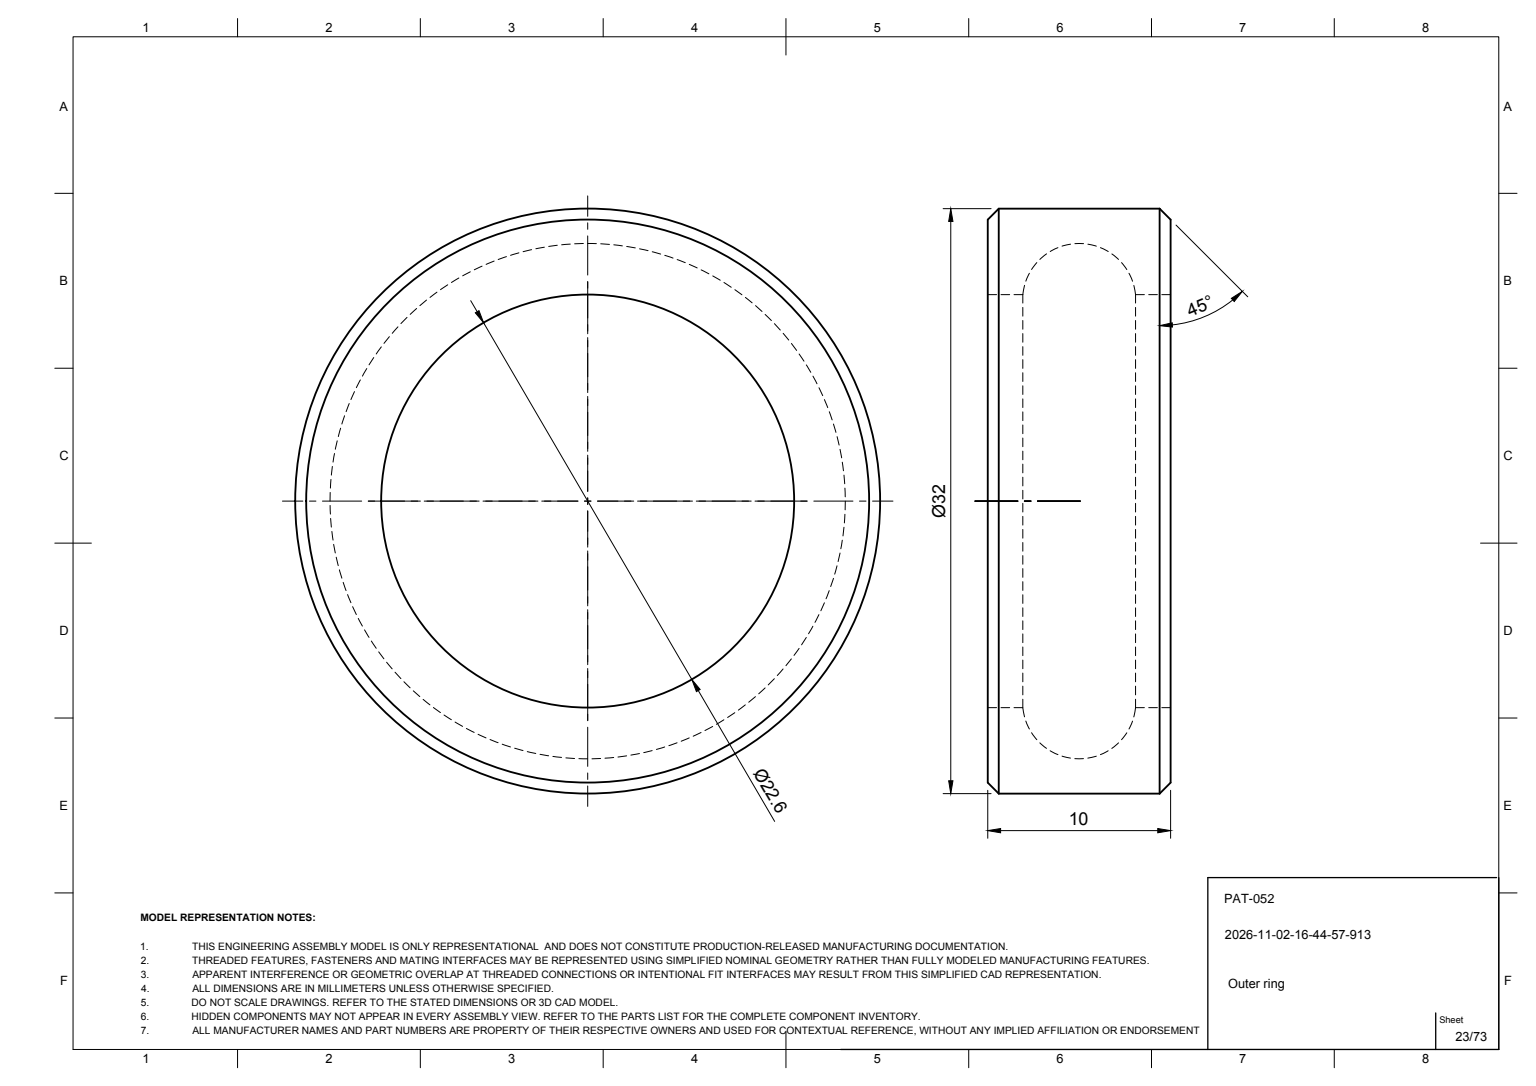
ISO-10303-21;
HEADER;
/* Generated by software containing ST-Developer
 * from STEP Tools, Inc. (www.steptools.com) 
 */

FILE_DESCRIPTION(
/* description */ ('Hand-crank gear train demonstrator'),
/* implementation_level */ '2;1');

FILE_NAME(
/* name */ 'Outer ring.step',
/* time_stamp */ '2026-10-28T03:22:13-07:00',
/* author */ (''),
/* organization */ (''),
/* preprocessor_version */ 'ST-DEVELOPER v20.2',
/* originating_system */ 'Autodesk Translation Framework v15.17.0.0',
/* authorisation */ '');

FILE_SCHEMA (('AUTOMOTIVE_DESIGN { 1 0 10303 214 3 1 1 }'));
ENDSEC;

DATA;
#10=MECHANICAL_DESIGN_GEOMETRIC_PRESENTATION_REPRESENTATION('',(#1201),#62758);
#1022=TOROIDAL_SURFACE('',#17506,1.1,0.309556);
#1030=CONICAL_SURFACE('',#17517,1.57,0.785398163397449);
#1031=CONICAL_SURFACE('',#17521,1.57,0.785398163397449);
#1073=SHAPE_REPRESENTATION_RELATIONSHIP('SRR','None',#63046,#1137);
#1137=ADVANCED_BREP_SHAPE_REPRESENTATION('',(#1279),#62700);
#1201=STYLED_ITEM('',(#63462),#1279);
#1279=MANIFOLD_SOLID_BREP('Body1',#16382);
#1489=FACE_BOUND('',#3355,.T.);
#1490=FACE_BOUND('',#3360,.T.);
#1684=PLANE('',#17514);
#1685=PLANE('',#17523);
#2269=FACE_OUTER_BOUND('',#3352,.T.);
#2270=FACE_OUTER_BOUND('',#3353,.T.);
#2271=FACE_OUTER_BOUND('',#3354,.T.);
#2272=FACE_OUTER_BOUND('',#3356,.T.);
#2273=FACE_OUTER_BOUND('',#3357,.T.);
#2274=FACE_OUTER_BOUND('',#3358,.T.);
#2275=FACE_OUTER_BOUND('',#3359,.T.);
#2276=FACE_OUTER_BOUND('',#3361,.T.);
#3352=EDGE_LOOP('',(#11491,#11492,#11493,#11494,#11495,#11496));
#3353=EDGE_LOOP('',(#11497,#11498,#11499,#11500,#11501));
#3354=EDGE_LOOP('',(#11502));
#3355=EDGE_LOOP('',(#11503));
#3356=EDGE_LOOP('',(#11504,#11505,#11506,#11507));
#3357=EDGE_LOOP('',(#11508,#11509,#11510,#11511));
#3358=EDGE_LOOP('',(#11512,#11513,#11514,#11515));
#3359=EDGE_LOOP('',(#11516));
#3360=EDGE_LOOP('',(#11517));
#3361=EDGE_LOOP('',(#11518,#11519,#11520,#11521,#11522));
#4428=LINE('',#24029,#5560);
#4429=LINE('',#24038,#5561);
#4430=LINE('',#24042,#5562);
#4431=LINE('',#24046,#5563);
#4432=LINE('',#24049,#5564);
#5560=VECTOR('',#19685,1.129765);
#5561=VECTOR('',#19696,1.57);
#5562=VECTOR('',#19701,1.6);
#5563=VECTOR('',#19706,1.57);
#5564=VECTOR('',#19711,1.129765);
#6736=CIRCLE('',#17507,1.129765);
#6737=CIRCLE('',#17508,1.129765);
#6738=CIRCLE('',#17509,0.309556);
#6739=CIRCLE('',#17510,1.129765);
#6740=CIRCLE('',#17511,1.129765);
#6741=CIRCLE('',#17513,1.129765);
#6742=CIRCLE('',#17515,1.54);
#6743=CIRCLE('',#17516,1.129765);
#6744=CIRCLE('',#17518,1.6);
#6745=CIRCLE('',#17520,1.6);
#6746=CIRCLE('',#17522,1.54);
#7429=VERTEX_POINT('',#24017);
#7430=VERTEX_POINT('',#24018);
#7431=VERTEX_POINT('',#24021);
#7432=VERTEX_POINT('',#24023);
#7433=VERTEX_POINT('',#24027);
#7434=VERTEX_POINT('',#24031);
#7435=VERTEX_POINT('',#24033);
#7436=VERTEX_POINT('',#24036);
#7437=VERTEX_POINT('',#24040);
#7438=VERTEX_POINT('',#24044);
#8997=EDGE_CURVE('',#7429,#7430,#6736,.T.);
#8998=EDGE_CURVE('',#7430,#7429,#6737,.T.);
#8999=EDGE_CURVE('',#7430,#7431,#6738,.T.);
#9000=EDGE_CURVE('',#7432,#7431,#6739,.T.);
#9001=EDGE_CURVE('',#7431,#7432,#6740,.T.);
#9002=EDGE_CURVE('',#7433,#7433,#6741,.T.);
#9003=EDGE_CURVE('',#7433,#7432,#4428,.T.);
#9004=EDGE_CURVE('',#7434,#7434,#6742,.T.);
#9005=EDGE_CURVE('',#7435,#7435,#6743,.T.);
#9006=EDGE_CURVE('',#7436,#7436,#6744,.T.);
#9007=EDGE_CURVE('',#7436,#7434,#4429,.T.);
#9008=EDGE_CURVE('',#7437,#7437,#6745,.T.);
#9009=EDGE_CURVE('',#7437,#7436,#4430,.T.);
#9010=EDGE_CURVE('',#7438,#7438,#6746,.T.);
#9011=EDGE_CURVE('',#7438,#7437,#4431,.T.);
#9012=EDGE_CURVE('',#7429,#7435,#4432,.T.);
#11491=ORIENTED_EDGE('',*,*,#8997,.F.);
#11492=ORIENTED_EDGE('',*,*,#8998,.F.);
#11493=ORIENTED_EDGE('',*,*,#8999,.T.);
#11494=ORIENTED_EDGE('',*,*,#9000,.F.);
#11495=ORIENTED_EDGE('',*,*,#9001,.F.);
#11496=ORIENTED_EDGE('',*,*,#8999,.F.);
#11497=ORIENTED_EDGE('',*,*,#9002,.T.);
#11498=ORIENTED_EDGE('',*,*,#9003,.T.);
#11499=ORIENTED_EDGE('',*,*,#9000,.T.);
#11500=ORIENTED_EDGE('',*,*,#9001,.T.);
#11501=ORIENTED_EDGE('',*,*,#9003,.F.);
#11502=ORIENTED_EDGE('',*,*,#9004,.F.);
#11503=ORIENTED_EDGE('',*,*,#9005,.T.);
#11504=ORIENTED_EDGE('',*,*,#9006,.F.);
#11505=ORIENTED_EDGE('',*,*,#9007,.T.);
#11506=ORIENTED_EDGE('',*,*,#9004,.T.);
#11507=ORIENTED_EDGE('',*,*,#9007,.F.);
#11508=ORIENTED_EDGE('',*,*,#9008,.F.);
#11509=ORIENTED_EDGE('',*,*,#9009,.T.);
#11510=ORIENTED_EDGE('',*,*,#9006,.T.);
#11511=ORIENTED_EDGE('',*,*,#9009,.F.);
#11512=ORIENTED_EDGE('',*,*,#9010,.F.);
#11513=ORIENTED_EDGE('',*,*,#9011,.T.);
#11514=ORIENTED_EDGE('',*,*,#9008,.T.);
#11515=ORIENTED_EDGE('',*,*,#9011,.F.);
#11516=ORIENTED_EDGE('',*,*,#9010,.T.);
#11517=ORIENTED_EDGE('',*,*,#9002,.F.);
#11518=ORIENTED_EDGE('',*,*,#8997,.T.);
#11519=ORIENTED_EDGE('',*,*,#8998,.T.);
#11520=ORIENTED_EDGE('',*,*,#9012,.T.);
#11521=ORIENTED_EDGE('',*,*,#9005,.F.);
#11522=ORIENTED_EDGE('',*,*,#9012,.F.);
#15256=CYLINDRICAL_SURFACE('',#17512,1.129765);
#15257=CYLINDRICAL_SURFACE('',#17519,1.6);
#15258=CYLINDRICAL_SURFACE('',#17524,1.129765);
#15579=ADVANCED_FACE('',(#2269),#1022,.F.);
#15580=ADVANCED_FACE('',(#2270),#15256,.F.);
#15581=ADVANCED_FACE('',(#2271,#1489),#1684,.T.);
#15582=ADVANCED_FACE('',(#2272),#1030,.T.);
#15583=ADVANCED_FACE('',(#2273),#15257,.T.);
#15584=ADVANCED_FACE('',(#2274),#1031,.T.);
#15585=ADVANCED_FACE('',(#2275,#1490),#1685,.T.);
#15586=ADVANCED_FACE('',(#2276),#15258,.F.);
#16382=CLOSED_SHELL('',(#15579,#15580,#15581,#15582,#15583,#15584,#15585,
#15586));
#17505=AXIS2_PLACEMENT_3D('',#24015,#19667,#19668);
#17506=AXIS2_PLACEMENT_3D('',#24016,#19669,#19670);
#17507=AXIS2_PLACEMENT_3D('',#24019,#19671,#19672);
#17508=AXIS2_PLACEMENT_3D('',#24020,#19673,#19674);
#17509=AXIS2_PLACEMENT_3D('',#24022,#19675,#19676);
#17510=AXIS2_PLACEMENT_3D('',#24024,#19677,#19678);
#17511=AXIS2_PLACEMENT_3D('',#24025,#19679,#19680);
#17512=AXIS2_PLACEMENT_3D('',#24026,#19681,#19682);
#17513=AXIS2_PLACEMENT_3D('',#24028,#19683,#19684);
#17514=AXIS2_PLACEMENT_3D('',#24030,#19686,#19687);
#17515=AXIS2_PLACEMENT_3D('',#24032,#19688,#19689);
#17516=AXIS2_PLACEMENT_3D('',#24034,#19690,#19691);
#17517=AXIS2_PLACEMENT_3D('',#24035,#19692,#19693);
#17518=AXIS2_PLACEMENT_3D('',#24037,#19694,#19695);
#17519=AXIS2_PLACEMENT_3D('',#24039,#19697,#19698);
#17520=AXIS2_PLACEMENT_3D('',#24041,#19699,#19700);
#17521=AXIS2_PLACEMENT_3D('',#24043,#19702,#19703);
#17522=AXIS2_PLACEMENT_3D('',#24045,#19704,#19705);
#17523=AXIS2_PLACEMENT_3D('',#24047,#19707,#19708);
#17524=AXIS2_PLACEMENT_3D('',#24048,#19709,#19710);
#19667=DIRECTION('axis',(0.,0.,1.));
#19668=DIRECTION('refdir',(1.,0.,0.));
#19669=DIRECTION('center_axis',(0.,-1.,0.));
#19670=DIRECTION('ref_axis',(0.,0.,-1.));
#19671=DIRECTION('center_axis',(0.,-1.,0.));
#19672=DIRECTION('ref_axis',(1.,0.,0.));
#19673=DIRECTION('center_axis',(0.,-1.,0.));
#19674=DIRECTION('ref_axis',(1.,0.,0.));
#19675=DIRECTION('center_axis',(1.,0.,1.22464679914735E-16));
#19676=DIRECTION('ref_axis',(-1.22464679914735E-16,0.,1.));
#19677=DIRECTION('center_axis',(0.,1.,0.));
#19678=DIRECTION('ref_axis',(1.,0.,0.));
#19679=DIRECTION('center_axis',(0.,1.,0.));
#19680=DIRECTION('ref_axis',(1.,0.,0.));
#19681=DIRECTION('center_axis',(0.,-1.,0.));
#19682=DIRECTION('ref_axis',(1.,0.,0.));
#19683=DIRECTION('center_axis',(0.,-1.,0.));
#19684=DIRECTION('ref_axis',(1.,0.,0.));
#19685=DIRECTION('',(0.,1.,0.));
#19686=DIRECTION('center_axis',(0.,1.,0.));
#19687=DIRECTION('ref_axis',(0.,0.,1.));
#19688=DIRECTION('center_axis',(0.,-1.,0.));
#19689=DIRECTION('ref_axis',(1.,0.,0.));
#19690=DIRECTION('center_axis',(0.,-1.,0.));
#19691=DIRECTION('ref_axis',(1.,0.,0.));
#19692=DIRECTION('center_axis',(0.,-1.,0.));
#19693=DIRECTION('ref_axis',(1.,0.,0.));
#19694=DIRECTION('center_axis',(0.,-1.,0.));
#19695=DIRECTION('ref_axis',(1.,0.,0.));
#19696=DIRECTION('',(0.707106781186548,0.707106781186547,8.65956056235494E-17));
#19697=DIRECTION('center_axis',(0.,-1.,0.));
#19698=DIRECTION('ref_axis',(1.,0.,0.));
#19699=DIRECTION('center_axis',(0.,-1.,0.));
#19700=DIRECTION('ref_axis',(1.,0.,0.));
#19701=DIRECTION('',(0.,1.,0.));
#19702=DIRECTION('center_axis',(0.,1.,0.));
#19703=DIRECTION('ref_axis',(1.,0.,0.));
#19704=DIRECTION('center_axis',(0.,-1.,0.));
#19705=DIRECTION('ref_axis',(1.,0.,0.));
#19706=DIRECTION('',(-0.707106781186548,0.707106781186547,-8.65956056235494E-17));
#19707=DIRECTION('center_axis',(0.,-1.,0.));
#19708=DIRECTION('ref_axis',(0.,0.,-1.));
#19709=DIRECTION('center_axis',(0.,-1.,0.));
#19710=DIRECTION('ref_axis',(1.,0.,0.));
#19711=DIRECTION('',(0.,1.,0.));
#24015=CARTESIAN_POINT('',(0.,0.,0.));
#24016=CARTESIAN_POINT('Origin',(0.,0.,0.));
#24017=CARTESIAN_POINT('',(-1.129765,0.308121667383195,-1.38356309103871E-16));
#24018=CARTESIAN_POINT('',(-1.38356309103871E-16,0.308121667383195,1.129765));
#24019=CARTESIAN_POINT('Origin',(0.,0.308121667383195,0.));
#24020=CARTESIAN_POINT('Origin',(0.,0.308121667383195,0.));
#24021=CARTESIAN_POINT('',(-1.38356309103871E-16,-0.308121667383195,1.129765));
#24022=CARTESIAN_POINT('Origin',(-1.34711147906209E-16,0.,1.1));
#24023=CARTESIAN_POINT('',(-1.129765,-0.308121667383195,1.38356309103871E-16));
#24024=CARTESIAN_POINT('Origin',(0.,-0.308121667383195,0.));
#24025=CARTESIAN_POINT('Origin',(0.,-0.308121667383195,0.));
#24026=CARTESIAN_POINT('Origin',(0.,0.,0.));
#24027=CARTESIAN_POINT('',(-1.129765,-0.5,-1.38356309103871E-16));
#24028=CARTESIAN_POINT('Origin',(0.,-0.5,0.));
#24029=CARTESIAN_POINT('',(-1.129765,0.,-1.38356309103871E-16));
#24030=CARTESIAN_POINT('Origin',(1.54,0.5,0.));
#24031=CARTESIAN_POINT('',(-1.54,0.5,-1.88595607068692E-16));
#24032=CARTESIAN_POINT('Origin',(0.,0.5,0.));
#24033=CARTESIAN_POINT('',(-1.129765,0.5,-1.38356309103871E-16));
#24034=CARTESIAN_POINT('Origin',(0.,0.5,0.));
#24035=CARTESIAN_POINT('Origin',(0.,0.47,0.));
#24036=CARTESIAN_POINT('',(-1.6,0.44,-1.95943487863577E-16));
#24037=CARTESIAN_POINT('Origin',(0.,0.44,0.));
#24038=CARTESIAN_POINT('',(-1.57,0.47,-1.92269547466134E-16));
#24039=CARTESIAN_POINT('Origin',(0.,0.,0.));
#24040=CARTESIAN_POINT('',(-1.6,-0.44,-1.95943487863577E-16));
#24041=CARTESIAN_POINT('Origin',(0.,-0.44,0.));
#24042=CARTESIAN_POINT('',(-1.6,0.,-1.95943487863577E-16));
#24043=CARTESIAN_POINT('Origin',(0.,-0.47,0.));
#24044=CARTESIAN_POINT('',(-1.54,-0.5,-1.88595607068692E-16));
#24045=CARTESIAN_POINT('Origin',(0.,-0.5,0.));
#24046=CARTESIAN_POINT('',(-1.57,-0.47,-1.92269547466134E-16));
#24047=CARTESIAN_POINT('Origin',(1.129765,-0.5,0.));
#24048=CARTESIAN_POINT('Origin',(0.,0.,0.));
#24049=CARTESIAN_POINT('',(-1.129765,0.,-1.38356309103871E-16));
#62626=UNCERTAINTY_MEASURE_WITH_UNIT(LENGTH_MEASURE(0.001),#62759,
'DISTANCE_ACCURACY_VALUE',
'Maximum model space distance between geometric entities at asserted c
onnectivities');
#62684=UNCERTAINTY_MEASURE_WITH_UNIT(LENGTH_MEASURE(0.001),#62759,
'DISTANCE_ACCURACY_VALUE',
'Maximum model space distance between geometric entities at asserted c
onnectivities');
#62700=(
GEOMETRIC_REPRESENTATION_CONTEXT(3)
GLOBAL_UNCERTAINTY_ASSIGNED_CONTEXT((#62626))
GLOBAL_UNIT_ASSIGNED_CONTEXT((#62759,#62761,#62762))
REPRESENTATION_CONTEXT('','3D')
);
#62758=(
GEOMETRIC_REPRESENTATION_CONTEXT(3)
GLOBAL_UNCERTAINTY_ASSIGNED_CONTEXT((#62684))
GLOBAL_UNIT_ASSIGNED_CONTEXT((#62759,#62761,#62762))
REPRESENTATION_CONTEXT('','3D')
);
#62759=(
LENGTH_UNIT()
NAMED_UNIT(*)
SI_UNIT(.CENTI.,.METRE.)
);
#62761=(
NAMED_UNIT(*)
PLANE_ANGLE_UNIT()
SI_UNIT($,.RADIAN.)
);
#62762=(
NAMED_UNIT(*)
SI_UNIT($,.STERADIAN.)
SOLID_ANGLE_UNIT()
);
#62778=SHAPE_DEFINITION_REPRESENTATION(#62851,#63046);
#62851=PRODUCT_DEFINITION_SHAPE('',$,#63120);
#63046=SHAPE_REPRESENTATION('',(#17505),#62700);
#63104=PRODUCT_DEFINITION_CONTEXT('part definition',#63325,'design');
#63120=PRODUCT_DEFINITION('Outer ring','Outer ring',#63193,#63104);
#63193=PRODUCT_DEFINITION_FORMATION('',$,#63342);
#63325=APPLICATION_CONTEXT(
'Core Data for Automotive Mechanical Design Process');
#63326=PRODUCT_CONTEXT('part definition',#63325,'mechanical');
#63342=PRODUCT('Outer ring','Outer ring','Outer ring',(#63326));
#63456=COLOUR_RGB('Grey',0.48,0.52,0.57);
#63457=FILL_AREA_STYLE_COLOUR('',#63456);
#63458=FILL_AREA_STYLE('',(#63457));
#63459=SURFACE_STYLE_FILL_AREA(#63458);
#63460=SURFACE_SIDE_STYLE('',(#63459));
#63461=SURFACE_STYLE_USAGE(.BOTH.,#63460);
#63462=PRESENTATION_STYLE_ASSIGNMENT((#63461));
ENDSEC;
END-ISO-10303-21;
